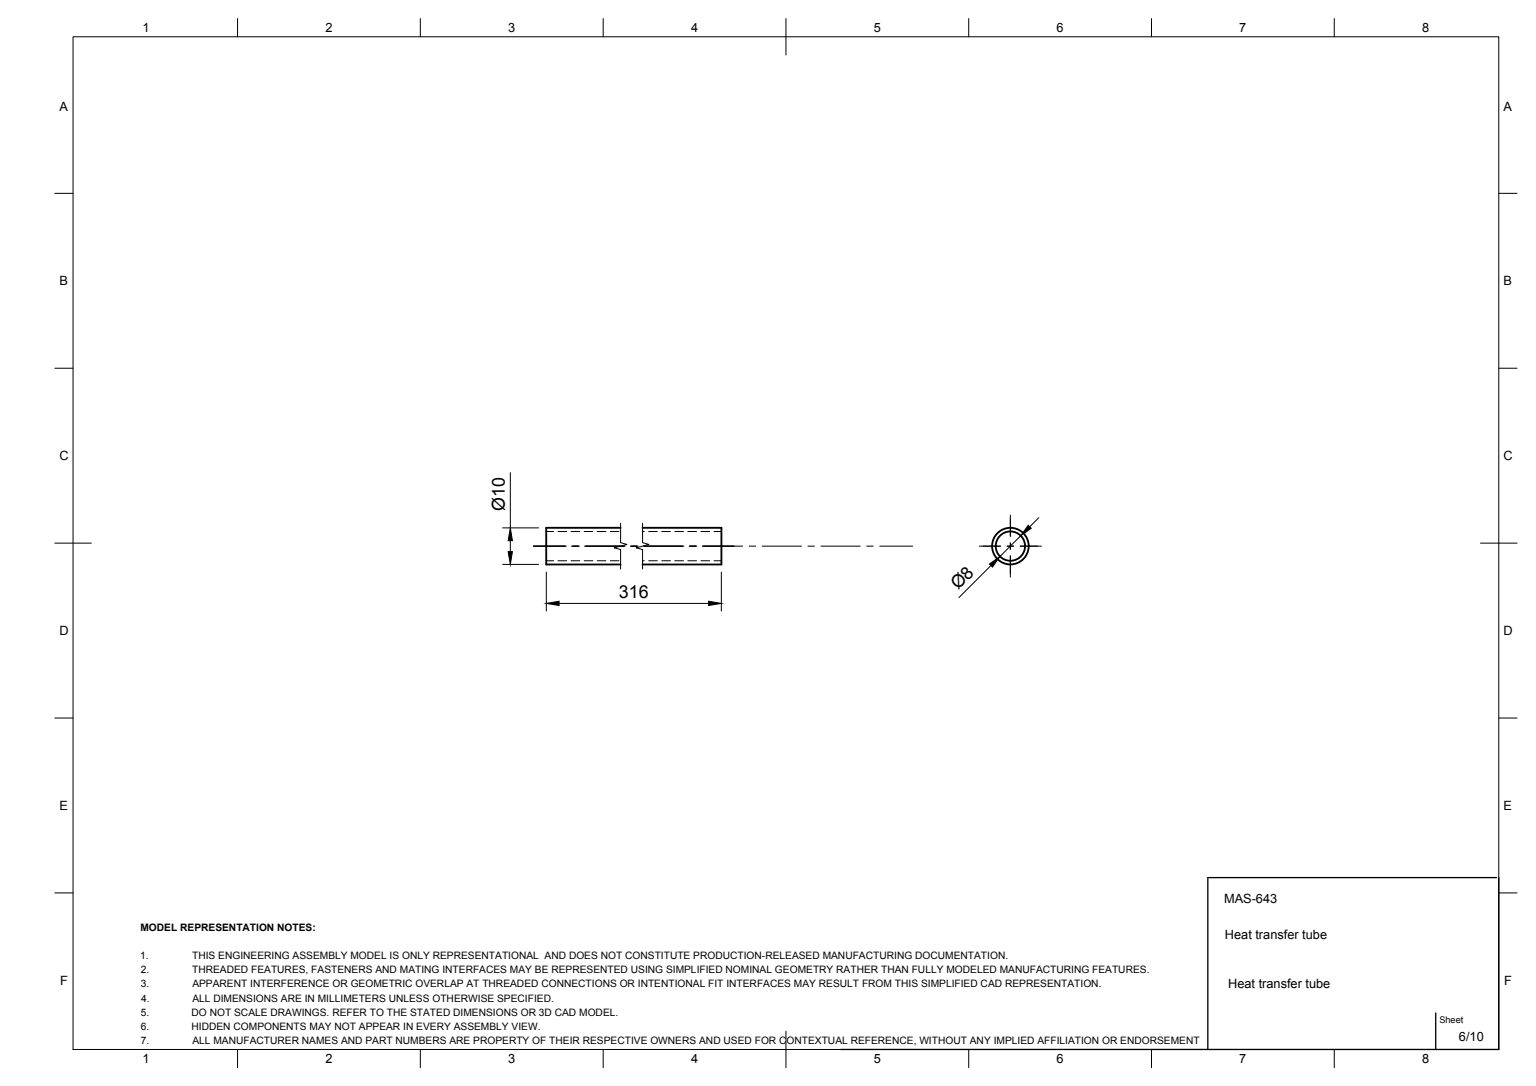
ISO-10303-21;
HEADER;
/* Generated by software containing ST-Developer
 * from STEP Tools, Inc. (www.steptools.com) 
 */

FILE_DESCRIPTION(
/* description */ ('Independent eighteen-tube parallel-flow evaporator geometry. Repeated
 machined headers and gasketed service covers, eighteen copper tubes, 
twenty-nine punched fins, threaded hose connections and bolted mountin
g feet. Native editable features and instanced parts. Braze details, w
orking fluid, pressure and thermal ratings require engineering selecti
on.'),
/* implementation_level */ '2;1');

FILE_NAME(
/* name */ 'Heat transfer tube.step',
/* time_stamp */ '2026-11-08T20:53:59-08:00',
/* author */ (''),
/* organization */ (''),
/* preprocessor_version */ 'ST-DEVELOPER v20.2',
/* originating_system */ 'Autodesk Translation Framework v15.17.0.0',
/* authorisation */ '');

FILE_SCHEMA (('AUTOMOTIVE_DESIGN { 1 0 10303 214 3 1 1 }'));
ENDSEC;

DATA;
#10=MECHANICAL_DESIGN_GEOMETRIC_PRESENTATION_REPRESENTATION('',(#336),#42620);
#316=SHAPE_REPRESENTATION_RELATIONSHIP('SRR','None',#42726,#326);
#326=ADVANCED_BREP_SHAPE_REPRESENTATION('',(#346),#42613);
#336=STYLED_ITEM('',(#42785),#346);
#346=MANIFOLD_SOLID_BREP('Body1',#10386);
#419=FACE_BOUND('',#1587,.T.);
#420=FACE_BOUND('',#1589,.T.);
#533=PLANE('',#10970);
#534=PLANE('',#10971);
#974=FACE_OUTER_BOUND('',#1584,.T.);
#975=FACE_OUTER_BOUND('',#1585,.T.);
#976=FACE_OUTER_BOUND('',#1586,.T.);
#977=FACE_OUTER_BOUND('',#1588,.T.);
#1584=EDGE_LOOP('',(#8531,#8532,#8533,#8534));
#1585=EDGE_LOOP('',(#8535,#8536,#8537,#8538));
#1586=EDGE_LOOP('',(#8539));
#1587=EDGE_LOOP('',(#8540));
#1588=EDGE_LOOP('',(#8541));
#1589=EDGE_LOOP('',(#8542));
#1927=CIRCLE('',#10965,4.);
#1928=CIRCLE('',#10966,4.);
#1929=CIRCLE('',#10968,5.);
#1930=CIRCLE('',#10969,5.);
#3162=LINE('',#34969,#3700);
#3163=LINE('',#34975,#3701);
#3700=VECTOR('',#12593,4.);
#3701=VECTOR('',#12600,5.);
#4583=VERTEX_POINT('',#34966);
#4584=VERTEX_POINT('',#34968);
#4585=VERTEX_POINT('',#34972);
#4586=VERTEX_POINT('',#34974);
#5948=EDGE_CURVE('',#4583,#4583,#1927,.T.);
#5949=EDGE_CURVE('',#4583,#4584,#3162,.T.);
#5950=EDGE_CURVE('',#4584,#4584,#1928,.T.);
#5951=EDGE_CURVE('',#4585,#4585,#1929,.T.);
#5952=EDGE_CURVE('',#4585,#4586,#3163,.T.);
#5953=EDGE_CURVE('',#4586,#4586,#1930,.T.);
#8531=ORIENTED_EDGE('',*,*,#5948,.F.);
#8532=ORIENTED_EDGE('',*,*,#5949,.T.);
#8533=ORIENTED_EDGE('',*,*,#5950,.T.);
#8534=ORIENTED_EDGE('',*,*,#5949,.F.);
#8535=ORIENTED_EDGE('',*,*,#5951,.F.);
#8536=ORIENTED_EDGE('',*,*,#5952,.T.);
#8537=ORIENTED_EDGE('',*,*,#5953,.T.);
#8538=ORIENTED_EDGE('',*,*,#5952,.F.);
#8539=ORIENTED_EDGE('',*,*,#5951,.T.);
#8540=ORIENTED_EDGE('',*,*,#5948,.T.);
#8541=ORIENTED_EDGE('',*,*,#5953,.F.);
#8542=ORIENTED_EDGE('',*,*,#5950,.F.);
#9720=CYLINDRICAL_SURFACE('',#10964,4.);
#9721=CYLINDRICAL_SURFACE('',#10967,5.);
#10210=ADVANCED_FACE('',(#974),#9720,.F.);
#10211=ADVANCED_FACE('',(#975),#9721,.T.);
#10212=ADVANCED_FACE('',(#976,#419),#533,.T.);
#10213=ADVANCED_FACE('',(#977,#420),#534,.F.);
#10386=CLOSED_SHELL('',(#10210,#10211,#10212,#10213));
#10963=AXIS2_PLACEMENT_3D('',#34964,#12587,#12588);
#10964=AXIS2_PLACEMENT_3D('',#34965,#12589,#12590);
#10965=AXIS2_PLACEMENT_3D('',#34967,#12591,#12592);
#10966=AXIS2_PLACEMENT_3D('',#34970,#12594,#12595);
#10967=AXIS2_PLACEMENT_3D('',#34971,#12596,#12597);
#10968=AXIS2_PLACEMENT_3D('',#34973,#12598,#12599);
#10969=AXIS2_PLACEMENT_3D('',#34976,#12601,#12602);
#10970=AXIS2_PLACEMENT_3D('',#34977,#12603,#12604);
#10971=AXIS2_PLACEMENT_3D('',#34978,#12605,#12606);
#12587=DIRECTION('axis',(0.,0.,1.));
#12588=DIRECTION('refdir',(1.,0.,0.));
#12589=DIRECTION('center_axis',(0.,0.,1.));
#12590=DIRECTION('ref_axis',(1.,0.,0.));
#12591=DIRECTION('center_axis',(0.,0.,-1.));
#12592=DIRECTION('ref_axis',(1.,0.,0.));
#12593=DIRECTION('',(0.,0.,-1.));
#12594=DIRECTION('center_axis',(0.,0.,-1.));
#12595=DIRECTION('ref_axis',(1.,0.,0.));
#12596=DIRECTION('center_axis',(0.,0.,1.));
#12597=DIRECTION('ref_axis',(1.,0.,0.));
#12598=DIRECTION('center_axis',(0.,0.,1.));
#12599=DIRECTION('ref_axis',(1.,0.,0.));
#12600=DIRECTION('',(0.,0.,-1.));
#12601=DIRECTION('center_axis',(0.,0.,1.));
#12602=DIRECTION('ref_axis',(1.,0.,0.));
#12603=DIRECTION('center_axis',(0.,0.,1.));
#12604=DIRECTION('ref_axis',(1.,0.,0.));
#12605=DIRECTION('center_axis',(0.,0.,1.));
#12606=DIRECTION('ref_axis',(1.,0.,0.));
#34964=CARTESIAN_POINT('',(0.,0.,0.));
#34965=CARTESIAN_POINT('Origin',(0.,0.,0.));
#34966=CARTESIAN_POINT('',(-4.,-4.89858719658941E-16,316.));
#34967=CARTESIAN_POINT('Origin',(0.,0.,316.));
#34968=CARTESIAN_POINT('',(-4.,-4.89858719658941E-16,0.));
#34969=CARTESIAN_POINT('',(-4.,-4.89858719658941E-16,0.));
#34970=CARTESIAN_POINT('Origin',(0.,0.,0.));
#34971=CARTESIAN_POINT('Origin',(0.,0.,0.));
#34972=CARTESIAN_POINT('',(-5.,-6.12323399573677E-16,316.));
#34973=CARTESIAN_POINT('Origin',(0.,0.,316.));
#34974=CARTESIAN_POINT('',(-5.,-6.12323399573677E-16,0.));
#34975=CARTESIAN_POINT('',(-5.,-6.12323399573677E-16,0.));
#34976=CARTESIAN_POINT('Origin',(0.,0.,0.));
#34977=CARTESIAN_POINT('Origin',(0.,0.,316.));
#34978=CARTESIAN_POINT('Origin',(0.,0.,0.));
#42601=UNCERTAINTY_MEASURE_WITH_UNIT(LENGTH_MEASURE(0.01),#42621,
'DISTANCE_ACCURACY_VALUE',
'Maximum model space distance between geometric entities at asserted c
onnectivities');
#42608=UNCERTAINTY_MEASURE_WITH_UNIT(LENGTH_MEASURE(0.01),#42621,
'DISTANCE_ACCURACY_VALUE',
'Maximum model space distance between geometric entities at asserted c
onnectivities');
#42613=(
GEOMETRIC_REPRESENTATION_CONTEXT(3)
GLOBAL_UNCERTAINTY_ASSIGNED_CONTEXT((#42601))
GLOBAL_UNIT_ASSIGNED_CONTEXT((#42621,#42623,#42624))
REPRESENTATION_CONTEXT('','3D')
);
#42620=(
GEOMETRIC_REPRESENTATION_CONTEXT(3)
GLOBAL_UNCERTAINTY_ASSIGNED_CONTEXT((#42608))
GLOBAL_UNIT_ASSIGNED_CONTEXT((#42621,#42623,#42624))
REPRESENTATION_CONTEXT('','3D')
);
#42621=(
LENGTH_UNIT()
NAMED_UNIT(*)
SI_UNIT(.MILLI.,.METRE.)
);
#42623=(
NAMED_UNIT(*)
PLANE_ANGLE_UNIT()
SI_UNIT($,.RADIAN.)
);
#42624=(
NAMED_UNIT(*)
SI_UNIT($,.STERADIAN.)
SOLID_ANGLE_UNIT()
);
#42629=SHAPE_DEFINITION_REPRESENTATION(#42640,#42726);
#42640=PRODUCT_DEFINITION_SHAPE('',$,#42738);
#42726=SHAPE_REPRESENTATION('',(#10963),#42613);
#42733=PRODUCT_DEFINITION_CONTEXT('part definition',#42768,'design');
#42738=PRODUCT_DEFINITION('Heat transfer tube','Heat transfer tube',#42749,
#42733);
#42749=PRODUCT_DEFINITION_FORMATION('',$,#42774);
#42768=APPLICATION_CONTEXT(
'Core Data for Automotive Mechanical Design Process');
#42769=PRODUCT_CONTEXT('part definition',#42768,'mechanical');
#42774=PRODUCT('Heat transfer tube','Heat transfer tube',$,(#42769));
#42785=PRESENTATION_STYLE_ASSIGNMENT((#42793));
#42793=SURFACE_STYLE_USAGE(.BOTH.,#42801);
#42801=SURFACE_SIDE_STYLE('',(#42809));
#42809=SURFACE_STYLE_FILL_AREA(#42817);
#42817=FILL_AREA_STYLE('Light blue',(#42825));
#42825=FILL_AREA_STYLE_COLOUR('Light blue',#42833);
#42833=COLOUR_RGB('Light blue',0.662745098039216,0.831372549019608,0.949019607843137);
ENDSEC;
END-ISO-10303-21;
